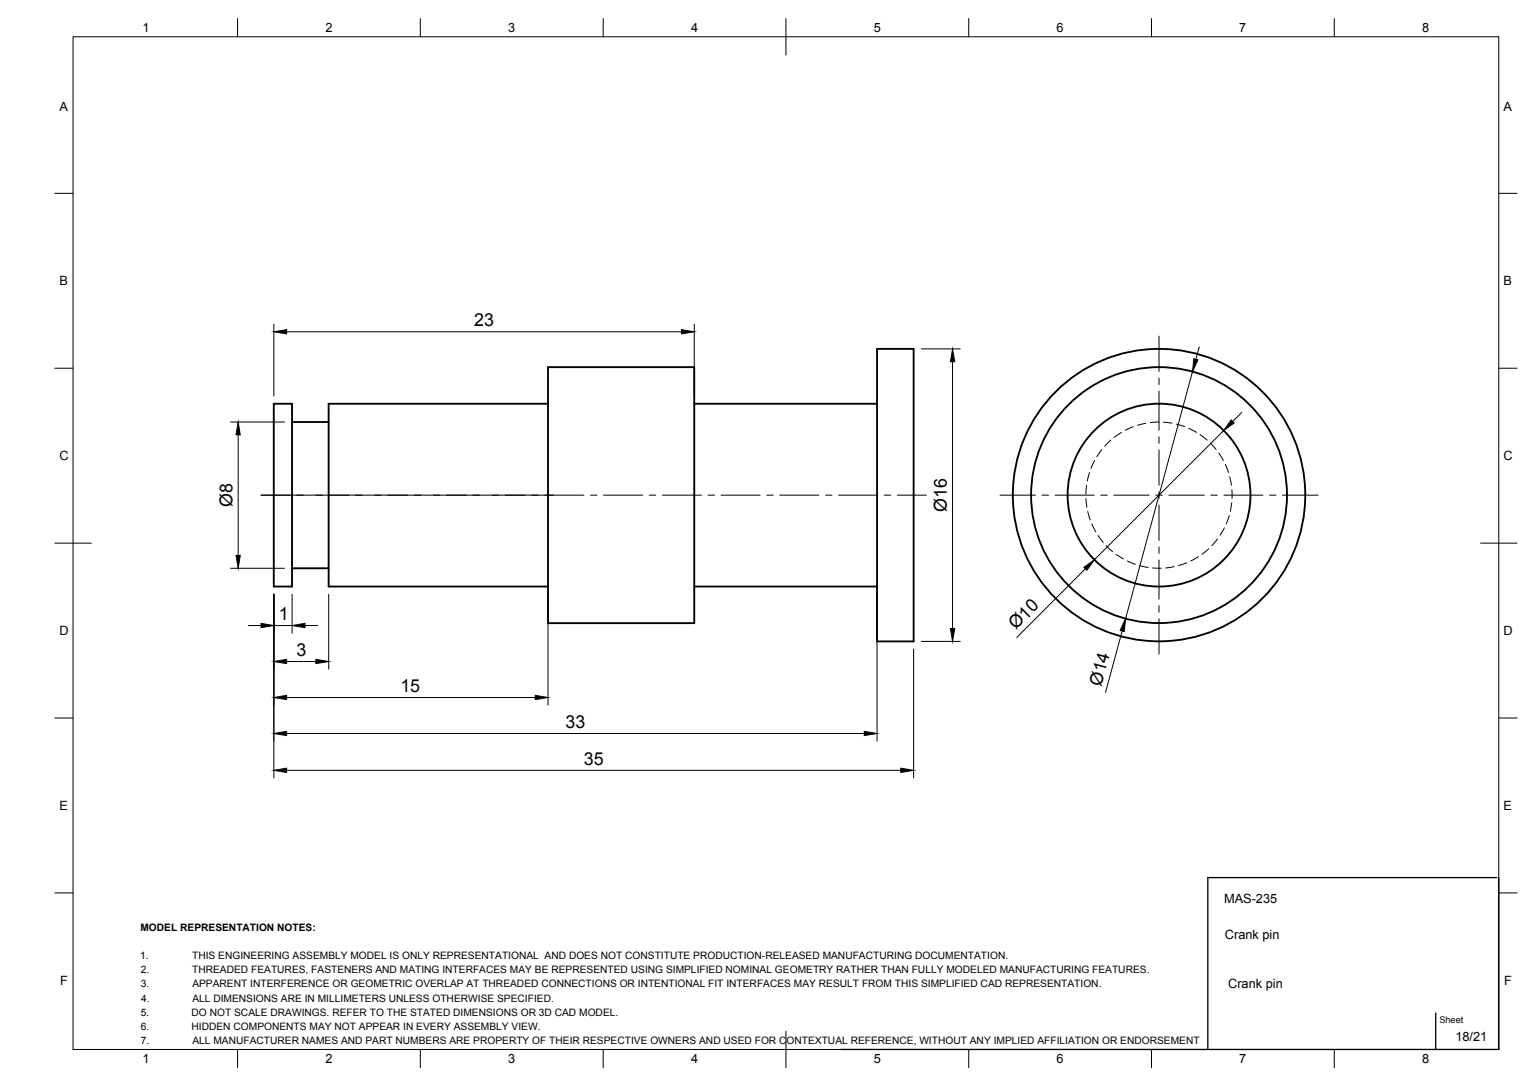
ISO-10303-21;
HEADER;
/* Generated by software containing ST-Developer
 * from STEP Tools, Inc. (www.steptools.com) 
 */

FILE_DESCRIPTION(
/* description */ ('Independent Whitworth quick-return mechanism. Crank radius40, ground-
center spacing80, lever180, connecting rod160, output guide X200. Nomi
nal stroke180 and long/short phase ratio2. Retained guide rods, replac
eable bearing sleeves and captured sliding shoe. No load or production
 rating assigned.'),
/* implementation_level */ '2;1');

FILE_NAME(
/* name */ 'Crank pin.step',
/* time_stamp */ '2026-11-09T18:22:56-08:00',
/* author */ (''),
/* organization */ (''),
/* preprocessor_version */ 'ST-DEVELOPER v20.2',
/* originating_system */ 'Autodesk Translation Framework v15.17.0.0',
/* authorisation */ '');

FILE_SCHEMA (('AUTOMOTIVE_DESIGN { 1 0 10303 214 3 1 1 }'));
ENDSEC;

DATA;
#10=MECHANICAL_DESIGN_GEOMETRIC_PRESENTATION_REPRESENTATION('',(#232),#4388);
#192=SHAPE_REPRESENTATION_RELATIONSHIP('SRR','None',#4491,#212);
#212=ADVANCED_BREP_SHAPE_REPRESENTATION('',(#252),#4381);
#232=STYLED_ITEM('',(#4595),#252);
#252=MANIFOLD_SOLID_BREP('Body1',#2337);
#302=FACE_BOUND('',#694,.T.);
#303=FACE_BOUND('',#696,.T.);
#304=FACE_BOUND('',#701,.T.);
#305=FACE_BOUND('',#703,.T.);
#306=FACE_BOUND('',#706,.T.);
#378=PLANE('',#2756);
#379=PLANE('',#2759);
#380=PLANE('',#2768);
#381=PLANE('',#2770);
#382=PLANE('',#2774);
#383=PLANE('',#2778);
#384=PLANE('',#2780);
#503=FACE_OUTER_BOUND('',#693,.T.);
#504=FACE_OUTER_BOUND('',#695,.T.);
#505=FACE_OUTER_BOUND('',#697,.T.);
#506=FACE_OUTER_BOUND('',#698,.T.);
#507=FACE_OUTER_BOUND('',#699,.T.);
#508=FACE_OUTER_BOUND('',#700,.T.);
#509=FACE_OUTER_BOUND('',#702,.T.);
#510=FACE_OUTER_BOUND('',#704,.T.);
#511=FACE_OUTER_BOUND('',#705,.T.);
#512=FACE_OUTER_BOUND('',#707,.T.);
#513=FACE_OUTER_BOUND('',#708,.T.);
#514=FACE_OUTER_BOUND('',#709,.T.);
#515=FACE_OUTER_BOUND('',#710,.T.);
#693=EDGE_LOOP('',(#1972));
#694=EDGE_LOOP('',(#1973));
#695=EDGE_LOOP('',(#1974));
#696=EDGE_LOOP('',(#1975));
#697=EDGE_LOOP('',(#1976,#1977,#1978,#1979));
#698=EDGE_LOOP('',(#1980,#1981,#1982,#1983));
#699=EDGE_LOOP('',(#1984,#1985,#1986,#1987));
#700=EDGE_LOOP('',(#1988));
#701=EDGE_LOOP('',(#1989));
#702=EDGE_LOOP('',(#1990));
#703=EDGE_LOOP('',(#1991));
#704=EDGE_LOOP('',(#1992,#1993,#1994,#1995));
#705=EDGE_LOOP('',(#1996));
#706=EDGE_LOOP('',(#1997));
#707=EDGE_LOOP('',(#1998,#1999,#2000,#2001));
#708=EDGE_LOOP('',(#2002));
#709=EDGE_LOOP('',(#2003,#2004,#2005,#2006));
#710=EDGE_LOOP('',(#2007));
#870=LINE('',#4139,#1009);
#871=LINE('',#4142,#1010);
#872=LINE('',#4148,#1011);
#873=LINE('',#4159,#1012);
#874=LINE('',#4165,#1013);
#875=LINE('',#4169,#1014);
#1009=VECTOR('',#3404,7.);
#1010=VECTOR('',#3407,5.);
#1011=VECTOR('',#3414,4.);
#1012=VECTOR('',#3429,5.);
#1013=VECTOR('',#3436,8.);
#1014=VECTOR('',#3443,5.);
#1115=CIRCLE('',#2757,7.);
#1116=CIRCLE('',#2758,5.);
#1117=CIRCLE('',#2760,7.);
#1118=CIRCLE('',#2761,5.);
#1119=CIRCLE('',#2764,5.);
#1120=CIRCLE('',#2766,4.);
#1121=CIRCLE('',#2767,4.);
#1122=CIRCLE('',#2769,5.);
#1123=CIRCLE('',#2771,5.);
#1124=CIRCLE('',#2773,5.);
#1125=CIRCLE('',#2775,8.);
#1126=CIRCLE('',#2777,8.);
#1285=VERTEX_POINT('',#4129);
#1286=VERTEX_POINT('',#4131);
#1287=VERTEX_POINT('',#4134);
#1288=VERTEX_POINT('',#4136);
#1289=VERTEX_POINT('',#4141);
#1290=VERTEX_POINT('',#4145);
#1291=VERTEX_POINT('',#4147);
#1292=VERTEX_POINT('',#4151);
#1293=VERTEX_POINT('',#4154);
#1294=VERTEX_POINT('',#4157);
#1295=VERTEX_POINT('',#4161);
#1296=VERTEX_POINT('',#4164);
#1522=EDGE_CURVE('',#1285,#1285,#1115,.T.);
#1523=EDGE_CURVE('',#1286,#1286,#1116,.T.);
#1524=EDGE_CURVE('',#1287,#1287,#1117,.T.);
#1525=EDGE_CURVE('',#1288,#1288,#1118,.T.);
#1526=EDGE_CURVE('',#1285,#1287,#870,.T.);
#1527=EDGE_CURVE('',#1288,#1289,#871,.T.);
#1528=EDGE_CURVE('',#1289,#1289,#1119,.T.);
#1529=EDGE_CURVE('',#1290,#1290,#1120,.T.);
#1530=EDGE_CURVE('',#1290,#1291,#872,.T.);
#1531=EDGE_CURVE('',#1291,#1291,#1121,.T.);
#1532=EDGE_CURVE('',#1292,#1292,#1122,.T.);
#1533=EDGE_CURVE('',#1293,#1293,#1123,.T.);
#1534=EDGE_CURVE('',#1294,#1294,#1124,.T.);
#1535=EDGE_CURVE('',#1294,#1293,#873,.T.);
#1536=EDGE_CURVE('',#1295,#1295,#1125,.T.);
#1537=EDGE_CURVE('',#1295,#1296,#874,.T.);
#1538=EDGE_CURVE('',#1296,#1296,#1126,.T.);
#1539=EDGE_CURVE('',#1292,#1286,#875,.T.);
#1972=ORIENTED_EDGE('',*,*,#1522,.T.);
#1973=ORIENTED_EDGE('',*,*,#1523,.F.);
#1974=ORIENTED_EDGE('',*,*,#1524,.F.);
#1975=ORIENTED_EDGE('',*,*,#1525,.F.);
#1976=ORIENTED_EDGE('',*,*,#1522,.F.);
#1977=ORIENTED_EDGE('',*,*,#1526,.T.);
#1978=ORIENTED_EDGE('',*,*,#1524,.T.);
#1979=ORIENTED_EDGE('',*,*,#1526,.F.);
#1980=ORIENTED_EDGE('',*,*,#1525,.T.);
#1981=ORIENTED_EDGE('',*,*,#1527,.T.);
#1982=ORIENTED_EDGE('',*,*,#1528,.T.);
#1983=ORIENTED_EDGE('',*,*,#1527,.F.);
#1984=ORIENTED_EDGE('',*,*,#1529,.T.);
#1985=ORIENTED_EDGE('',*,*,#1530,.T.);
#1986=ORIENTED_EDGE('',*,*,#1531,.F.);
#1987=ORIENTED_EDGE('',*,*,#1530,.F.);
#1988=ORIENTED_EDGE('',*,*,#1532,.F.);
#1989=ORIENTED_EDGE('',*,*,#1529,.F.);
#1990=ORIENTED_EDGE('',*,*,#1533,.F.);
#1991=ORIENTED_EDGE('',*,*,#1531,.T.);
#1992=ORIENTED_EDGE('',*,*,#1534,.F.);
#1993=ORIENTED_EDGE('',*,*,#1535,.T.);
#1994=ORIENTED_EDGE('',*,*,#1533,.T.);
#1995=ORIENTED_EDGE('',*,*,#1535,.F.);
#1996=ORIENTED_EDGE('',*,*,#1536,.T.);
#1997=ORIENTED_EDGE('',*,*,#1528,.F.);
#1998=ORIENTED_EDGE('',*,*,#1536,.F.);
#1999=ORIENTED_EDGE('',*,*,#1537,.T.);
#2000=ORIENTED_EDGE('',*,*,#1538,.T.);
#2001=ORIENTED_EDGE('',*,*,#1537,.F.);
#2002=ORIENTED_EDGE('',*,*,#1538,.F.);
#2003=ORIENTED_EDGE('',*,*,#1532,.T.);
#2004=ORIENTED_EDGE('',*,*,#1539,.T.);
#2005=ORIENTED_EDGE('',*,*,#1523,.T.);
#2006=ORIENTED_EDGE('',*,*,#1539,.F.);
#2007=ORIENTED_EDGE('',*,*,#1534,.T.);
#2155=CYLINDRICAL_SURFACE('',#2762,7.);
#2156=CYLINDRICAL_SURFACE('',#2763,5.);
#2157=CYLINDRICAL_SURFACE('',#2765,4.);
#2158=CYLINDRICAL_SURFACE('',#2772,5.);
#2159=CYLINDRICAL_SURFACE('',#2776,8.);
#2160=CYLINDRICAL_SURFACE('',#2779,5.);
#2275=ADVANCED_FACE('',(#503,#302),#378,.T.);
#2276=ADVANCED_FACE('',(#504,#303),#379,.F.);
#2277=ADVANCED_FACE('',(#505),#2155,.T.);
#2278=ADVANCED_FACE('',(#506),#2156,.T.);
#2279=ADVANCED_FACE('',(#507),#2157,.T.);
#2280=ADVANCED_FACE('',(#508,#304),#380,.F.);
#2281=ADVANCED_FACE('',(#509,#305),#381,.F.);
#2282=ADVANCED_FACE('',(#510),#2158,.T.);
#2283=ADVANCED_FACE('',(#511,#306),#382,.T.);
#2284=ADVANCED_FACE('',(#512),#2159,.T.);
#2285=ADVANCED_FACE('',(#513),#383,.F.);
#2286=ADVANCED_FACE('',(#514),#2160,.T.);
#2287=ADVANCED_FACE('',(#515),#384,.T.);
#2337=CLOSED_SHELL('',(#2275,#2276,#2277,#2278,#2279,#2280,#2281,#2282,
#2283,#2284,#2285,#2286,#2287));
#2755=AXIS2_PLACEMENT_3D('',#4127,#3388,#3389);
#2756=AXIS2_PLACEMENT_3D('',#4128,#3390,#3391);
#2757=AXIS2_PLACEMENT_3D('',#4130,#3392,#3393);
#2758=AXIS2_PLACEMENT_3D('',#4132,#3394,#3395);
#2759=AXIS2_PLACEMENT_3D('',#4133,#3396,#3397);
#2760=AXIS2_PLACEMENT_3D('',#4135,#3398,#3399);
#2761=AXIS2_PLACEMENT_3D('',#4137,#3400,#3401);
#2762=AXIS2_PLACEMENT_3D('',#4138,#3402,#3403);
#2763=AXIS2_PLACEMENT_3D('',#4140,#3405,#3406);
#2764=AXIS2_PLACEMENT_3D('',#4143,#3408,#3409);
#2765=AXIS2_PLACEMENT_3D('',#4144,#3410,#3411);
#2766=AXIS2_PLACEMENT_3D('',#4146,#3412,#3413);
#2767=AXIS2_PLACEMENT_3D('',#4149,#3415,#3416);
#2768=AXIS2_PLACEMENT_3D('',#4150,#3417,#3418);
#2769=AXIS2_PLACEMENT_3D('',#4152,#3419,#3420);
#2770=AXIS2_PLACEMENT_3D('',#4153,#3421,#3422);
#2771=AXIS2_PLACEMENT_3D('',#4155,#3423,#3424);
#2772=AXIS2_PLACEMENT_3D('',#4156,#3425,#3426);
#2773=AXIS2_PLACEMENT_3D('',#4158,#3427,#3428);
#2774=AXIS2_PLACEMENT_3D('',#4160,#3430,#3431);
#2775=AXIS2_PLACEMENT_3D('',#4162,#3432,#3433);
#2776=AXIS2_PLACEMENT_3D('',#4163,#3434,#3435);
#2777=AXIS2_PLACEMENT_3D('',#4166,#3437,#3438);
#2778=AXIS2_PLACEMENT_3D('',#4167,#3439,#3440);
#2779=AXIS2_PLACEMENT_3D('',#4168,#3441,#3442);
#2780=AXIS2_PLACEMENT_3D('',#4170,#3444,#3445);
#3388=DIRECTION('axis',(0.,0.,1.));
#3389=DIRECTION('refdir',(1.,0.,0.));
#3390=DIRECTION('center_axis',(0.,0.,1.));
#3391=DIRECTION('ref_axis',(1.,0.,0.));
#3392=DIRECTION('center_axis',(0.,0.,1.));
#3393=DIRECTION('ref_axis',(1.,0.,0.));
#3394=DIRECTION('center_axis',(0.,0.,1.));
#3395=DIRECTION('ref_axis',(1.,0.,0.));
#3396=DIRECTION('center_axis',(0.,0.,1.));
#3397=DIRECTION('ref_axis',(1.,0.,0.));
#3398=DIRECTION('center_axis',(0.,0.,1.));
#3399=DIRECTION('ref_axis',(1.,0.,0.));
#3400=DIRECTION('center_axis',(0.,0.,-1.));
#3401=DIRECTION('ref_axis',(1.,0.,0.));
#3402=DIRECTION('center_axis',(0.,0.,1.));
#3403=DIRECTION('ref_axis',(1.,0.,0.));
#3404=DIRECTION('',(0.,0.,-1.));
#3405=DIRECTION('center_axis',(0.,0.,1.));
#3406=DIRECTION('ref_axis',(1.,0.,0.));
#3407=DIRECTION('',(0.,0.,-1.));
#3408=DIRECTION('center_axis',(0.,0.,1.));
#3409=DIRECTION('ref_axis',(1.,0.,0.));
#3410=DIRECTION('center_axis',(0.,0.,1.));
#3411=DIRECTION('ref_axis',(1.,0.,0.));
#3412=DIRECTION('center_axis',(0.,0.,1.));
#3413=DIRECTION('ref_axis',(1.,0.,0.));
#3414=DIRECTION('',(0.,0.,1.));
#3415=DIRECTION('center_axis',(0.,0.,1.));
#3416=DIRECTION('ref_axis',(1.,0.,0.));
#3417=DIRECTION('center_axis',(0.,0.,-1.));
#3418=DIRECTION('ref_axis',(-1.,0.,0.));
#3419=DIRECTION('center_axis',(0.,0.,-1.));
#3420=DIRECTION('ref_axis',(1.,0.,0.));
#3421=DIRECTION('center_axis',(0.,0.,1.));
#3422=DIRECTION('ref_axis',(1.,0.,0.));
#3423=DIRECTION('center_axis',(0.,0.,1.));
#3424=DIRECTION('ref_axis',(1.,0.,0.));
#3425=DIRECTION('center_axis',(0.,0.,1.));
#3426=DIRECTION('ref_axis',(1.,0.,0.));
#3427=DIRECTION('center_axis',(0.,0.,1.));
#3428=DIRECTION('ref_axis',(1.,0.,0.));
#3429=DIRECTION('',(0.,0.,-1.));
#3430=DIRECTION('center_axis',(0.,0.,1.));
#3431=DIRECTION('ref_axis',(1.,0.,0.));
#3432=DIRECTION('center_axis',(0.,0.,1.));
#3433=DIRECTION('ref_axis',(1.,0.,0.));
#3434=DIRECTION('center_axis',(0.,0.,1.));
#3435=DIRECTION('ref_axis',(1.,0.,0.));
#3436=DIRECTION('',(0.,0.,-1.));
#3437=DIRECTION('center_axis',(0.,0.,1.));
#3438=DIRECTION('ref_axis',(1.,0.,0.));
#3439=DIRECTION('center_axis',(0.,0.,1.));
#3440=DIRECTION('ref_axis',(1.,0.,0.));
#3441=DIRECTION('center_axis',(0.,0.,1.));
#3442=DIRECTION('ref_axis',(1.,0.,0.));
#3443=DIRECTION('',(0.,0.,-1.));
#3444=DIRECTION('center_axis',(0.,0.,1.));
#3445=DIRECTION('ref_axis',(1.,0.,0.));
#4127=CARTESIAN_POINT('',(0.,0.,0.));
#4128=CARTESIAN_POINT('Origin',(0.,0.,18.));
#4129=CARTESIAN_POINT('',(-7.,-8.57252759403147E-16,18.));
#4130=CARTESIAN_POINT('Origin',(0.,0.,18.));
#4131=CARTESIAN_POINT('',(-5.,-6.12323399573677E-16,18.));
#4132=CARTESIAN_POINT('Origin',(0.,0.,18.));
#4133=CARTESIAN_POINT('Origin',(0.,0.,10.));
#4134=CARTESIAN_POINT('',(-7.,-8.57252759403147E-16,10.));
#4135=CARTESIAN_POINT('Origin',(0.,0.,10.));
#4136=CARTESIAN_POINT('',(-5.,6.12323399573677E-16,10.));
#4137=CARTESIAN_POINT('Origin',(0.,0.,10.));
#4138=CARTESIAN_POINT('Origin',(0.,0.,10.));
#4139=CARTESIAN_POINT('',(-7.,-8.57252759403147E-16,10.));
#4140=CARTESIAN_POINT('Origin',(0.,0.,0.));
#4141=CARTESIAN_POINT('',(-5.,-6.12323399573677E-16,0.));
#4142=CARTESIAN_POINT('',(-5.,-6.12323399573677E-16,0.));
#4143=CARTESIAN_POINT('Origin',(0.,0.,0.));
#4144=CARTESIAN_POINT('Origin',(0.,0.,31.));
#4145=CARTESIAN_POINT('',(-4.,-4.89858719658941E-16,30.));
#4146=CARTESIAN_POINT('Origin',(0.,0.,30.));
#4147=CARTESIAN_POINT('',(-4.,-4.89858719658941E-16,32.));
#4148=CARTESIAN_POINT('',(-4.,-4.89858719658941E-16,31.));
#4149=CARTESIAN_POINT('Origin',(0.,0.,32.));
#4150=CARTESIAN_POINT('Origin',(8.,0.,30.));
#4151=CARTESIAN_POINT('',(-5.,6.12323399573677E-16,30.));
#4152=CARTESIAN_POINT('Origin',(0.,0.,30.));
#4153=CARTESIAN_POINT('Origin',(4.,0.,32.));
#4154=CARTESIAN_POINT('',(-5.,-6.12323399573677E-16,32.));
#4155=CARTESIAN_POINT('Origin',(0.,0.,32.));
#4156=CARTESIAN_POINT('Origin',(0.,0.,0.));
#4157=CARTESIAN_POINT('',(-5.,-6.12323399573677E-16,33.));
#4158=CARTESIAN_POINT('Origin',(0.,0.,33.));
#4159=CARTESIAN_POINT('',(-5.,-6.12323399573677E-16,0.));
#4160=CARTESIAN_POINT('Origin',(0.,0.,0.));
#4161=CARTESIAN_POINT('',(-8.,-9.79717439317883E-16,0.));
#4162=CARTESIAN_POINT('Origin',(0.,0.,0.));
#4163=CARTESIAN_POINT('Origin',(0.,0.,-2.));
#4164=CARTESIAN_POINT('',(-8.,-9.79717439317883E-16,-2.));
#4165=CARTESIAN_POINT('',(-8.,-9.79717439317883E-16,-2.));
#4166=CARTESIAN_POINT('Origin',(0.,0.,-2.));
#4167=CARTESIAN_POINT('Origin',(0.,0.,-2.));
#4168=CARTESIAN_POINT('Origin',(0.,0.,0.));
#4169=CARTESIAN_POINT('',(-5.,-6.12323399573677E-16,0.));
#4170=CARTESIAN_POINT('Origin',(0.,0.,33.));
#4359=UNCERTAINTY_MEASURE_WITH_UNIT(LENGTH_MEASURE(0.01),#4389,
'DISTANCE_ACCURACY_VALUE',
'Maximum model space distance between geometric entities at asserted c
onnectivities');
#4366=UNCERTAINTY_MEASURE_WITH_UNIT(LENGTH_MEASURE(0.01),#4389,
'DISTANCE_ACCURACY_VALUE',
'Maximum model space distance between geometric entities at asserted c
onnectivities');
#4381=(
GEOMETRIC_REPRESENTATION_CONTEXT(3)
GLOBAL_UNCERTAINTY_ASSIGNED_CONTEXT((#4359))
GLOBAL_UNIT_ASSIGNED_CONTEXT((#4389,#4391,#4392))
REPRESENTATION_CONTEXT('','3D')
);
#4388=(
GEOMETRIC_REPRESENTATION_CONTEXT(3)
GLOBAL_UNCERTAINTY_ASSIGNED_CONTEXT((#4366))
GLOBAL_UNIT_ASSIGNED_CONTEXT((#4389,#4391,#4392))
REPRESENTATION_CONTEXT('','3D')
);
#4389=(
LENGTH_UNIT()
NAMED_UNIT(*)
SI_UNIT(.MILLI.,.METRE.)
);
#4391=(
NAMED_UNIT(*)
PLANE_ANGLE_UNIT()
SI_UNIT($,.RADIAN.)
);
#4392=(
NAMED_UNIT(*)
SI_UNIT($,.STERADIAN.)
SOLID_ANGLE_UNIT()
);
#4407=SHAPE_DEFINITION_REPRESENTATION(#4428,#4491);
#4428=PRODUCT_DEFINITION_SHAPE('',$,#4513);
#4491=SHAPE_REPRESENTATION('',(#2755),#4381);
#4498=PRODUCT_DEFINITION_CONTEXT('part definition',#4563,'design');
#4513=PRODUCT_DEFINITION('Crank pin','Crank pin',#4534,#4498);
#4534=PRODUCT_DEFINITION_FORMATION('',$,#4579);
#4563=APPLICATION_CONTEXT(
'Core Data for Automotive Mechanical Design Process');
#4564=PRODUCT_CONTEXT('part definition',#4563,'mechanical');
#4579=PRODUCT('Crank pin','Crank pin','Crank pin',(#4564));
#4595=PRESENTATION_STYLE_ASSIGNMENT((#4609));
#4609=SURFACE_STYLE_USAGE(.BOTH.,#4623);
#4623=SURFACE_SIDE_STYLE('',(#4637));
#4637=SURFACE_STYLE_FILL_AREA(#4651);
#4651=FILL_AREA_STYLE('Pivot gray',(#4665));
#4665=FILL_AREA_STYLE_COLOUR('Pivot gray',#4679);
#4679=COLOUR_RGB('Pivot gray',0.407843137254902,0.447058823529412,0.498039215686275);
ENDSEC;
END-ISO-10303-21;
